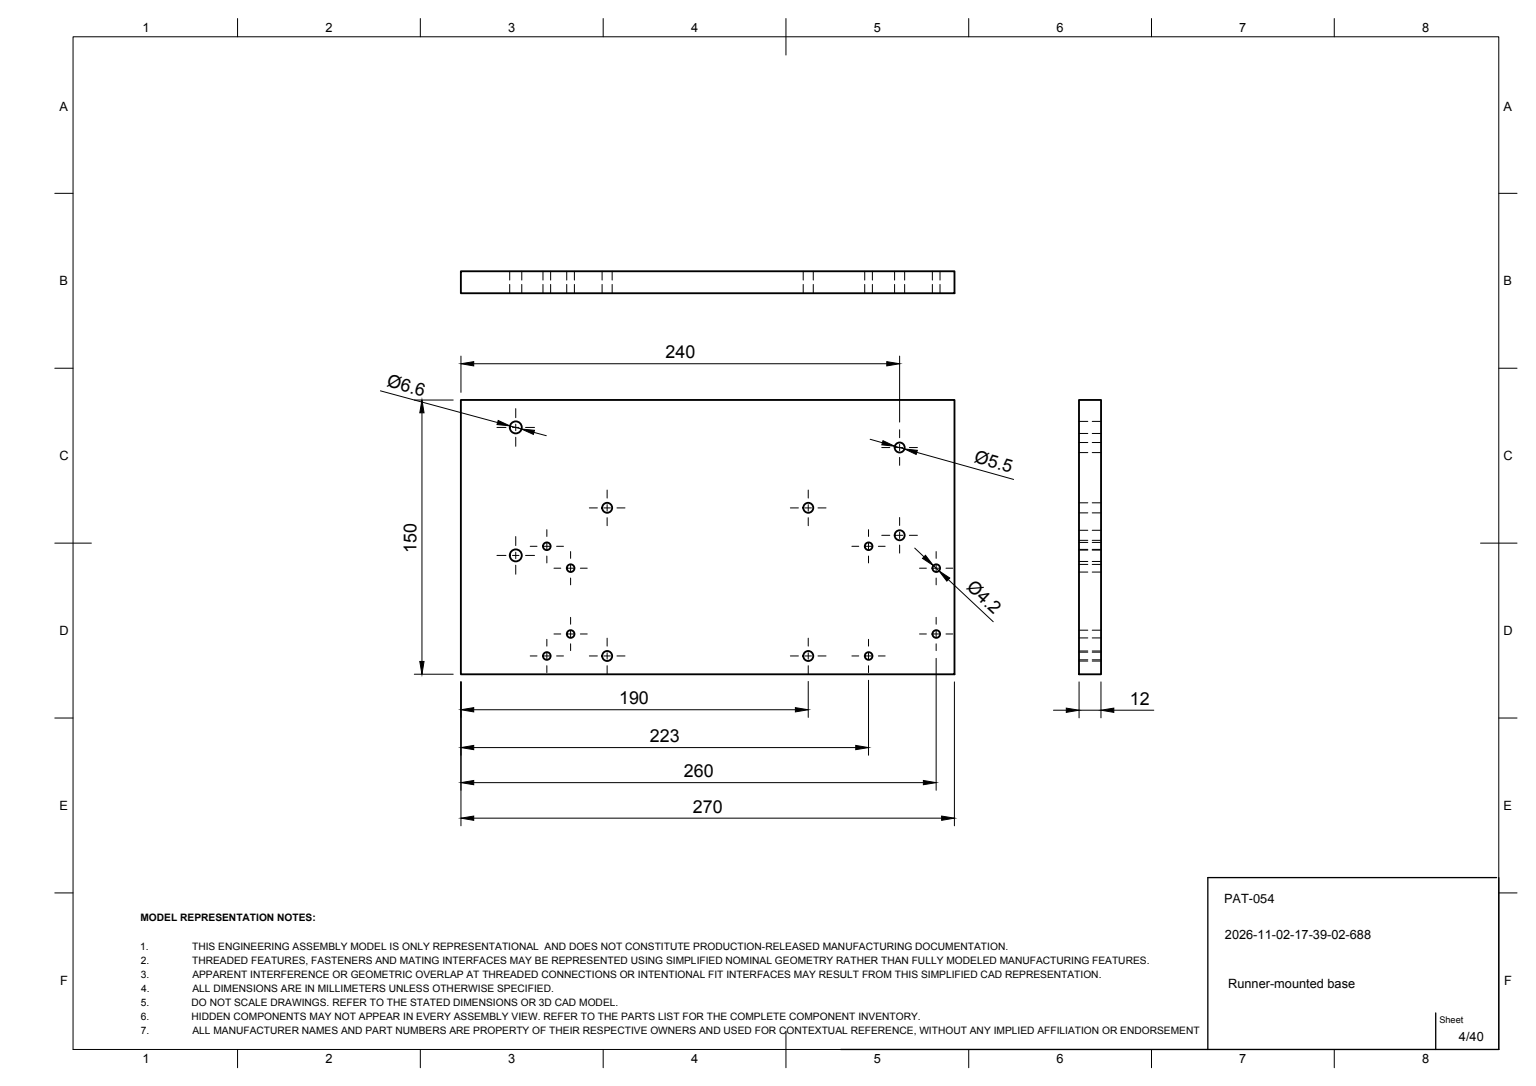
ISO-10303-21;
HEADER;
/* Generated by software containing ST-Developer
 * from STEP Tools, Inc. (www.steptools.com) 
 */

FILE_DESCRIPTION(
/* description */ ('PAT-054'),
/* implementation_level */ '2;1');

FILE_NAME(
/* name */ 'Runner-mounted base.step',
/* time_stamp */ '2026-10-29T16:38:13-07:00',
/* author */ (''),
/* organization */ (''),
/* preprocessor_version */ 'ST-DEVELOPER v20.2',
/* originating_system */ 'Autodesk Translation Framework v15.17.0.0',
/* authorisation */ '');

FILE_SCHEMA (('AUTOMOTIVE_DESIGN { 1 0 10303 214 3 1 1 }'));
ENDSEC;

DATA;
#10=MECHANICAL_DESIGN_GEOMETRIC_PRESENTATION_REPRESENTATION('',(#899),#33981);
#811=SHAPE_REPRESENTATION_RELATIONSHIP('SRR','None',#34184,#855);
#855=ADVANCED_BREP_SHAPE_REPRESENTATION('',(#958),#33932);
#899=STYLED_ITEM('',(#34496),#958);
#958=MANIFOLD_SOLID_BREP('Body1',#13010);
#1012=FACE_BOUND('',#2319,.T.);
#1013=FACE_BOUND('',#2320,.T.);
#1014=FACE_BOUND('',#2321,.T.);
#1015=FACE_BOUND('',#2322,.T.);
#1016=FACE_BOUND('',#2323,.T.);
#1017=FACE_BOUND('',#2324,.T.);
#1018=FACE_BOUND('',#2325,.T.);
#1019=FACE_BOUND('',#2326,.T.);
#1020=FACE_BOUND('',#2327,.T.);
#1021=FACE_BOUND('',#2328,.T.);
#1022=FACE_BOUND('',#2329,.T.);
#1023=FACE_BOUND('',#2330,.T.);
#1024=FACE_BOUND('',#2331,.T.);
#1025=FACE_BOUND('',#2332,.T.);
#1026=FACE_BOUND('',#2333,.T.);
#1027=FACE_BOUND('',#2334,.T.);
#1028=FACE_BOUND('',#2336,.T.);
#1029=FACE_BOUND('',#2337,.T.);
#1030=FACE_BOUND('',#2338,.T.);
#1031=FACE_BOUND('',#2339,.T.);
#1032=FACE_BOUND('',#2340,.T.);
#1033=FACE_BOUND('',#2341,.T.);
#1034=FACE_BOUND('',#2342,.T.);
#1035=FACE_BOUND('',#2343,.T.);
#1036=FACE_BOUND('',#2344,.T.);
#1037=FACE_BOUND('',#2345,.T.);
#1038=FACE_BOUND('',#2346,.T.);
#1039=FACE_BOUND('',#2347,.T.);
#1040=FACE_BOUND('',#2348,.T.);
#1041=FACE_BOUND('',#2349,.T.);
#1042=FACE_BOUND('',#2350,.T.);
#1043=FACE_BOUND('',#2351,.T.);
#1228=PLANE('',#13610);
#1229=PLANE('',#13611);
#1230=PLANE('',#13612);
#1231=PLANE('',#13613);
#1232=PLANE('',#13614);
#1233=PLANE('',#13615);
#1575=FACE_OUTER_BOUND('',#2298,.T.);
#1576=FACE_OUTER_BOUND('',#2299,.T.);
#1577=FACE_OUTER_BOUND('',#2300,.T.);
#1578=FACE_OUTER_BOUND('',#2301,.T.);
#1579=FACE_OUTER_BOUND('',#2302,.T.);
#1580=FACE_OUTER_BOUND('',#2303,.T.);
#1581=FACE_OUTER_BOUND('',#2304,.T.);
#1582=FACE_OUTER_BOUND('',#2305,.T.);
#1583=FACE_OUTER_BOUND('',#2306,.T.);
#1584=FACE_OUTER_BOUND('',#2307,.T.);
#1585=FACE_OUTER_BOUND('',#2308,.T.);
#1586=FACE_OUTER_BOUND('',#2309,.T.);
#1587=FACE_OUTER_BOUND('',#2310,.T.);
#1588=FACE_OUTER_BOUND('',#2311,.T.);
#1589=FACE_OUTER_BOUND('',#2312,.T.);
#1590=FACE_OUTER_BOUND('',#2313,.T.);
#1591=FACE_OUTER_BOUND('',#2314,.T.);
#1592=FACE_OUTER_BOUND('',#2315,.T.);
#1593=FACE_OUTER_BOUND('',#2316,.T.);
#1594=FACE_OUTER_BOUND('',#2317,.T.);
#1595=FACE_OUTER_BOUND('',#2318,.T.);
#1596=FACE_OUTER_BOUND('',#2335,.T.);
#2298=EDGE_LOOP('',(#8489,#8490,#8491,#8492));
#2299=EDGE_LOOP('',(#8493,#8494,#8495,#8496));
#2300=EDGE_LOOP('',(#8497,#8498,#8499,#8500));
#2301=EDGE_LOOP('',(#8501,#8502,#8503,#8504));
#2302=EDGE_LOOP('',(#8505,#8506,#8507,#8508));
#2303=EDGE_LOOP('',(#8509,#8510,#8511,#8512));
#2304=EDGE_LOOP('',(#8513,#8514,#8515,#8516));
#2305=EDGE_LOOP('',(#8517,#8518,#8519,#8520));
#2306=EDGE_LOOP('',(#8521,#8522,#8523,#8524));
#2307=EDGE_LOOP('',(#8525,#8526,#8527,#8528));
#2308=EDGE_LOOP('',(#8529,#8530,#8531,#8532));
#2309=EDGE_LOOP('',(#8533,#8534,#8535,#8536));
#2310=EDGE_LOOP('',(#8537,#8538,#8539,#8540));
#2311=EDGE_LOOP('',(#8541,#8542,#8543,#8544));
#2312=EDGE_LOOP('',(#8545,#8546,#8547,#8548));
#2313=EDGE_LOOP('',(#8549,#8550,#8551,#8552));
#2314=EDGE_LOOP('',(#8553,#8554,#8555,#8556));
#2315=EDGE_LOOP('',(#8557,#8558,#8559,#8560));
#2316=EDGE_LOOP('',(#8561,#8562,#8563,#8564));
#2317=EDGE_LOOP('',(#8565,#8566,#8567,#8568));
#2318=EDGE_LOOP('',(#8569,#8570,#8571,#8572));
#2319=EDGE_LOOP('',(#8573));
#2320=EDGE_LOOP('',(#8574));
#2321=EDGE_LOOP('',(#8575));
#2322=EDGE_LOOP('',(#8576));
#2323=EDGE_LOOP('',(#8577));
#2324=EDGE_LOOP('',(#8578));
#2325=EDGE_LOOP('',(#8579));
#2326=EDGE_LOOP('',(#8580));
#2327=EDGE_LOOP('',(#8581));
#2328=EDGE_LOOP('',(#8582));
#2329=EDGE_LOOP('',(#8583));
#2330=EDGE_LOOP('',(#8584));
#2331=EDGE_LOOP('',(#8585));
#2332=EDGE_LOOP('',(#8586));
#2333=EDGE_LOOP('',(#8587));
#2334=EDGE_LOOP('',(#8588));
#2335=EDGE_LOOP('',(#8589,#8590,#8591,#8592));
#2336=EDGE_LOOP('',(#8593));
#2337=EDGE_LOOP('',(#8594));
#2338=EDGE_LOOP('',(#8595));
#2339=EDGE_LOOP('',(#8596));
#2340=EDGE_LOOP('',(#8597));
#2341=EDGE_LOOP('',(#8598));
#2342=EDGE_LOOP('',(#8599));
#2343=EDGE_LOOP('',(#8600));
#2344=EDGE_LOOP('',(#8601));
#2345=EDGE_LOOP('',(#8602));
#2346=EDGE_LOOP('',(#8603));
#2347=EDGE_LOOP('',(#8604));
#2348=EDGE_LOOP('',(#8605));
#2349=EDGE_LOOP('',(#8606));
#2350=EDGE_LOOP('',(#8607));
#2351=EDGE_LOOP('',(#8608));
#3237=LINE('',#18493,#4171);
#3238=LINE('',#18499,#4172);
#3239=LINE('',#18505,#4173);
#3240=LINE('',#18511,#4174);
#3241=LINE('',#18517,#4175);
#3242=LINE('',#18523,#4176);
#3243=LINE('',#18529,#4177);
#3244=LINE('',#18535,#4178);
#3245=LINE('',#18541,#4179);
#3246=LINE('',#18547,#4180);
#3247=LINE('',#18553,#4181);
#3248=LINE('',#18559,#4182);
#3249=LINE('',#18565,#4183);
#3250=LINE('',#18571,#4184);
#3251=LINE('',#18577,#4185);
#3252=LINE('',#18583,#4186);
#3253=LINE('',#18588,#4187);
#3254=LINE('',#18590,#4188);
#3255=LINE('',#18592,#4189);
#3256=LINE('',#18593,#4190);
#3257=LINE('',#18596,#4191);
#3258=LINE('',#18598,#4192);
#3259=LINE('',#18599,#4193);
#3260=LINE('',#18602,#4194);
#3261=LINE('',#18604,#4195);
#3262=LINE('',#18605,#4196);
#3263=LINE('',#18607,#4197);
#3264=LINE('',#18608,#4198);
#4171=VECTOR('',#14900,0.274999999999999);
#4172=VECTOR('',#14907,0.275);
#4173=VECTOR('',#14914,0.275);
#4174=VECTOR('',#14921,0.274999999999999);
#4175=VECTOR('',#14928,0.210000000000001);
#4176=VECTOR('',#14935,0.210000000000001);
#4177=VECTOR('',#14942,0.21);
#4178=VECTOR('',#14949,0.21);
#4179=VECTOR('',#14956,0.329999999999998);
#4180=VECTOR('',#14963,0.329999999999998);
#4181=VECTOR('',#14970,0.275);
#4182=VECTOR('',#14977,0.275);
#4183=VECTOR('',#14984,0.210000000000001);
#4184=VECTOR('',#14991,0.21);
#4185=VECTOR('',#14998,0.21);
#4186=VECTOR('',#15005,0.210000000000001);
#4187=VECTOR('',#15010,1.);
#4188=VECTOR('',#15011,1.);
#4189=VECTOR('',#15012,1.);
#4190=VECTOR('',#15013,1.);
#4191=VECTOR('',#15016,1.);
#4192=VECTOR('',#15017,1.);
#4193=VECTOR('',#15018,1.);
#4194=VECTOR('',#15021,1.);
#4195=VECTOR('',#15022,1.);
#4196=VECTOR('',#15023,1.);
#4197=VECTOR('',#15026,1.);
#4198=VECTOR('',#15027,1.);
#5105=CIRCLE('',#13563,0.274999999999999);
#5106=CIRCLE('',#13564,0.274999999999999);
#5107=CIRCLE('',#13566,0.275);
#5108=CIRCLE('',#13567,0.275);
#5109=CIRCLE('',#13569,0.275);
#5110=CIRCLE('',#13570,0.275);
#5111=CIRCLE('',#13572,0.274999999999999);
#5112=CIRCLE('',#13573,0.274999999999999);
#5113=CIRCLE('',#13575,0.210000000000001);
#5114=CIRCLE('',#13576,0.210000000000001);
#5115=CIRCLE('',#13578,0.210000000000001);
#5116=CIRCLE('',#13579,0.210000000000001);
#5117=CIRCLE('',#13581,0.21);
#5118=CIRCLE('',#13582,0.21);
#5119=CIRCLE('',#13584,0.21);
#5120=CIRCLE('',#13585,0.21);
#5121=CIRCLE('',#13587,0.329999999999998);
#5122=CIRCLE('',#13588,0.329999999999998);
#5123=CIRCLE('',#13590,0.329999999999998);
#5124=CIRCLE('',#13591,0.329999999999998);
#5125=CIRCLE('',#13593,0.275);
#5126=CIRCLE('',#13594,0.275);
#5127=CIRCLE('',#13596,0.275);
#5128=CIRCLE('',#13597,0.275);
#5129=CIRCLE('',#13599,0.210000000000001);
#5130=CIRCLE('',#13600,0.210000000000001);
#5131=CIRCLE('',#13602,0.21);
#5132=CIRCLE('',#13603,0.21);
#5133=CIRCLE('',#13605,0.21);
#5134=CIRCLE('',#13606,0.21);
#5135=CIRCLE('',#13608,0.210000000000001);
#5136=CIRCLE('',#13609,0.210000000000001);
#5570=VERTEX_POINT('',#18490);
#5571=VERTEX_POINT('',#18492);
#5572=VERTEX_POINT('',#18496);
#5573=VERTEX_POINT('',#18498);
#5574=VERTEX_POINT('',#18502);
#5575=VERTEX_POINT('',#18504);
#5576=VERTEX_POINT('',#18508);
#5577=VERTEX_POINT('',#18510);
#5578=VERTEX_POINT('',#18514);
#5579=VERTEX_POINT('',#18516);
#5580=VERTEX_POINT('',#18520);
#5581=VERTEX_POINT('',#18522);
#5582=VERTEX_POINT('',#18526);
#5583=VERTEX_POINT('',#18528);
#5584=VERTEX_POINT('',#18532);
#5585=VERTEX_POINT('',#18534);
#5586=VERTEX_POINT('',#18538);
#5587=VERTEX_POINT('',#18540);
#5588=VERTEX_POINT('',#18544);
#5589=VERTEX_POINT('',#18546);
#5590=VERTEX_POINT('',#18550);
#5591=VERTEX_POINT('',#18552);
#5592=VERTEX_POINT('',#18556);
#5593=VERTEX_POINT('',#18558);
#5594=VERTEX_POINT('',#18562);
#5595=VERTEX_POINT('',#18564);
#5596=VERTEX_POINT('',#18568);
#5597=VERTEX_POINT('',#18570);
#5598=VERTEX_POINT('',#18574);
#5599=VERTEX_POINT('',#18576);
#5600=VERTEX_POINT('',#18580);
#5601=VERTEX_POINT('',#18582);
#5602=VERTEX_POINT('',#18586);
#5603=VERTEX_POINT('',#18587);
#5604=VERTEX_POINT('',#18589);
#5605=VERTEX_POINT('',#18591);
#5606=VERTEX_POINT('',#18595);
#5607=VERTEX_POINT('',#18597);
#5608=VERTEX_POINT('',#18601);
#5609=VERTEX_POINT('',#18603);
#6744=EDGE_CURVE('',#5570,#5570,#5105,.T.);
#6745=EDGE_CURVE('',#5570,#5571,#3237,.T.);
#6746=EDGE_CURVE('',#5571,#5571,#5106,.T.);
#6747=EDGE_CURVE('',#5572,#5572,#5107,.T.);
#6748=EDGE_CURVE('',#5572,#5573,#3238,.T.);
#6749=EDGE_CURVE('',#5573,#5573,#5108,.T.);
#6750=EDGE_CURVE('',#5574,#5574,#5109,.T.);
#6751=EDGE_CURVE('',#5574,#5575,#3239,.T.);
#6752=EDGE_CURVE('',#5575,#5575,#5110,.T.);
#6753=EDGE_CURVE('',#5576,#5576,#5111,.T.);
#6754=EDGE_CURVE('',#5576,#5577,#3240,.T.);
#6755=EDGE_CURVE('',#5577,#5577,#5112,.T.);
#6756=EDGE_CURVE('',#5578,#5578,#5113,.T.);
#6757=EDGE_CURVE('',#5578,#5579,#3241,.T.);
#6758=EDGE_CURVE('',#5579,#5579,#5114,.T.);
#6759=EDGE_CURVE('',#5580,#5580,#5115,.T.);
#6760=EDGE_CURVE('',#5580,#5581,#3242,.T.);
#6761=EDGE_CURVE('',#5581,#5581,#5116,.T.);
#6762=EDGE_CURVE('',#5582,#5582,#5117,.T.);
#6763=EDGE_CURVE('',#5582,#5583,#3243,.T.);
#6764=EDGE_CURVE('',#5583,#5583,#5118,.T.);
#6765=EDGE_CURVE('',#5584,#5584,#5119,.T.);
#6766=EDGE_CURVE('',#5584,#5585,#3244,.T.);
#6767=EDGE_CURVE('',#5585,#5585,#5120,.T.);
#6768=EDGE_CURVE('',#5586,#5586,#5121,.T.);
#6769=EDGE_CURVE('',#5586,#5587,#3245,.T.);
#6770=EDGE_CURVE('',#5587,#5587,#5122,.T.);
#6771=EDGE_CURVE('',#5588,#5588,#5123,.T.);
#6772=EDGE_CURVE('',#5588,#5589,#3246,.T.);
#6773=EDGE_CURVE('',#5589,#5589,#5124,.T.);
#6774=EDGE_CURVE('',#5590,#5590,#5125,.T.);
#6775=EDGE_CURVE('',#5590,#5591,#3247,.T.);
#6776=EDGE_CURVE('',#5591,#5591,#5126,.T.);
#6777=EDGE_CURVE('',#5592,#5592,#5127,.T.);
#6778=EDGE_CURVE('',#5592,#5593,#3248,.T.);
#6779=EDGE_CURVE('',#5593,#5593,#5128,.T.);
#6780=EDGE_CURVE('',#5594,#5594,#5129,.T.);
#6781=EDGE_CURVE('',#5594,#5595,#3249,.T.);
#6782=EDGE_CURVE('',#5595,#5595,#5130,.T.);
#6783=EDGE_CURVE('',#5596,#5596,#5131,.T.);
#6784=EDGE_CURVE('',#5596,#5597,#3250,.T.);
#6785=EDGE_CURVE('',#5597,#5597,#5132,.T.);
#6786=EDGE_CURVE('',#5598,#5598,#5133,.T.);
#6787=EDGE_CURVE('',#5598,#5599,#3251,.T.);
#6788=EDGE_CURVE('',#5599,#5599,#5134,.T.);
#6789=EDGE_CURVE('',#5600,#5600,#5135,.T.);
#6790=EDGE_CURVE('',#5600,#5601,#3252,.T.);
#6791=EDGE_CURVE('',#5601,#5601,#5136,.T.);
#6792=EDGE_CURVE('',#5602,#5603,#3253,.T.);
#6793=EDGE_CURVE('',#5603,#5604,#3254,.T.);
#6794=EDGE_CURVE('',#5605,#5604,#3255,.T.);
#6795=EDGE_CURVE('',#5602,#5605,#3256,.T.);
#6796=EDGE_CURVE('',#5606,#5602,#3257,.T.);
#6797=EDGE_CURVE('',#5607,#5605,#3258,.T.);
#6798=EDGE_CURVE('',#5606,#5607,#3259,.T.);
#6799=EDGE_CURVE('',#5608,#5606,#3260,.T.);
#6800=EDGE_CURVE('',#5609,#5607,#3261,.T.);
#6801=EDGE_CURVE('',#5608,#5609,#3262,.T.);
#6802=EDGE_CURVE('',#5603,#5608,#3263,.T.);
#6803=EDGE_CURVE('',#5604,#5609,#3264,.T.);
#8489=ORIENTED_EDGE('',*,*,#6744,.F.);
#8490=ORIENTED_EDGE('',*,*,#6745,.T.);
#8491=ORIENTED_EDGE('',*,*,#6746,.F.);
#8492=ORIENTED_EDGE('',*,*,#6745,.F.);
#8493=ORIENTED_EDGE('',*,*,#6747,.F.);
#8494=ORIENTED_EDGE('',*,*,#6748,.T.);
#8495=ORIENTED_EDGE('',*,*,#6749,.F.);
#8496=ORIENTED_EDGE('',*,*,#6748,.F.);
#8497=ORIENTED_EDGE('',*,*,#6750,.F.);
#8498=ORIENTED_EDGE('',*,*,#6751,.T.);
#8499=ORIENTED_EDGE('',*,*,#6752,.F.);
#8500=ORIENTED_EDGE('',*,*,#6751,.F.);
#8501=ORIENTED_EDGE('',*,*,#6753,.F.);
#8502=ORIENTED_EDGE('',*,*,#6754,.T.);
#8503=ORIENTED_EDGE('',*,*,#6755,.F.);
#8504=ORIENTED_EDGE('',*,*,#6754,.F.);
#8505=ORIENTED_EDGE('',*,*,#6756,.F.);
#8506=ORIENTED_EDGE('',*,*,#6757,.T.);
#8507=ORIENTED_EDGE('',*,*,#6758,.F.);
#8508=ORIENTED_EDGE('',*,*,#6757,.F.);
#8509=ORIENTED_EDGE('',*,*,#6759,.F.);
#8510=ORIENTED_EDGE('',*,*,#6760,.T.);
#8511=ORIENTED_EDGE('',*,*,#6761,.F.);
#8512=ORIENTED_EDGE('',*,*,#6760,.F.);
#8513=ORIENTED_EDGE('',*,*,#6762,.F.);
#8514=ORIENTED_EDGE('',*,*,#6763,.T.);
#8515=ORIENTED_EDGE('',*,*,#6764,.F.);
#8516=ORIENTED_EDGE('',*,*,#6763,.F.);
#8517=ORIENTED_EDGE('',*,*,#6765,.F.);
#8518=ORIENTED_EDGE('',*,*,#6766,.T.);
#8519=ORIENTED_EDGE('',*,*,#6767,.F.);
#8520=ORIENTED_EDGE('',*,*,#6766,.F.);
#8521=ORIENTED_EDGE('',*,*,#6768,.F.);
#8522=ORIENTED_EDGE('',*,*,#6769,.T.);
#8523=ORIENTED_EDGE('',*,*,#6770,.F.);
#8524=ORIENTED_EDGE('',*,*,#6769,.F.);
#8525=ORIENTED_EDGE('',*,*,#6771,.F.);
#8526=ORIENTED_EDGE('',*,*,#6772,.T.);
#8527=ORIENTED_EDGE('',*,*,#6773,.F.);
#8528=ORIENTED_EDGE('',*,*,#6772,.F.);
#8529=ORIENTED_EDGE('',*,*,#6774,.F.);
#8530=ORIENTED_EDGE('',*,*,#6775,.T.);
#8531=ORIENTED_EDGE('',*,*,#6776,.F.);
#8532=ORIENTED_EDGE('',*,*,#6775,.F.);
#8533=ORIENTED_EDGE('',*,*,#6777,.F.);
#8534=ORIENTED_EDGE('',*,*,#6778,.T.);
#8535=ORIENTED_EDGE('',*,*,#6779,.F.);
#8536=ORIENTED_EDGE('',*,*,#6778,.F.);
#8537=ORIENTED_EDGE('',*,*,#6780,.F.);
#8538=ORIENTED_EDGE('',*,*,#6781,.T.);
#8539=ORIENTED_EDGE('',*,*,#6782,.F.);
#8540=ORIENTED_EDGE('',*,*,#6781,.F.);
#8541=ORIENTED_EDGE('',*,*,#6783,.F.);
#8542=ORIENTED_EDGE('',*,*,#6784,.T.);
#8543=ORIENTED_EDGE('',*,*,#6785,.F.);
#8544=ORIENTED_EDGE('',*,*,#6784,.F.);
#8545=ORIENTED_EDGE('',*,*,#6786,.F.);
#8546=ORIENTED_EDGE('',*,*,#6787,.T.);
#8547=ORIENTED_EDGE('',*,*,#6788,.F.);
#8548=ORIENTED_EDGE('',*,*,#6787,.F.);
#8549=ORIENTED_EDGE('',*,*,#6789,.F.);
#8550=ORIENTED_EDGE('',*,*,#6790,.T.);
#8551=ORIENTED_EDGE('',*,*,#6791,.F.);
#8552=ORIENTED_EDGE('',*,*,#6790,.F.);
#8553=ORIENTED_EDGE('',*,*,#6792,.T.);
#8554=ORIENTED_EDGE('',*,*,#6793,.T.);
#8555=ORIENTED_EDGE('',*,*,#6794,.F.);
#8556=ORIENTED_EDGE('',*,*,#6795,.F.);
#8557=ORIENTED_EDGE('',*,*,#6796,.T.);
#8558=ORIENTED_EDGE('',*,*,#6795,.T.);
#8559=ORIENTED_EDGE('',*,*,#6797,.F.);
#8560=ORIENTED_EDGE('',*,*,#6798,.F.);
#8561=ORIENTED_EDGE('',*,*,#6799,.T.);
#8562=ORIENTED_EDGE('',*,*,#6798,.T.);
#8563=ORIENTED_EDGE('',*,*,#6800,.F.);
#8564=ORIENTED_EDGE('',*,*,#6801,.F.);
#8565=ORIENTED_EDGE('',*,*,#6802,.T.);
#8566=ORIENTED_EDGE('',*,*,#6801,.T.);
#8567=ORIENTED_EDGE('',*,*,#6803,.F.);
#8568=ORIENTED_EDGE('',*,*,#6793,.F.);
#8569=ORIENTED_EDGE('',*,*,#6803,.T.);
#8570=ORIENTED_EDGE('',*,*,#6800,.T.);
#8571=ORIENTED_EDGE('',*,*,#6797,.T.);
#8572=ORIENTED_EDGE('',*,*,#6794,.T.);
#8573=ORIENTED_EDGE('',*,*,#6758,.T.);
#8574=ORIENTED_EDGE('',*,*,#6761,.T.);
#8575=ORIENTED_EDGE('',*,*,#6770,.T.);
#8576=ORIENTED_EDGE('',*,*,#6773,.T.);
#8577=ORIENTED_EDGE('',*,*,#6776,.T.);
#8578=ORIENTED_EDGE('',*,*,#6779,.T.);
#8579=ORIENTED_EDGE('',*,*,#6782,.T.);
#8580=ORIENTED_EDGE('',*,*,#6785,.T.);
#8581=ORIENTED_EDGE('',*,*,#6788,.T.);
#8582=ORIENTED_EDGE('',*,*,#6791,.T.);
#8583=ORIENTED_EDGE('',*,*,#6767,.T.);
#8584=ORIENTED_EDGE('',*,*,#6764,.T.);
#8585=ORIENTED_EDGE('',*,*,#6755,.T.);
#8586=ORIENTED_EDGE('',*,*,#6752,.T.);
#8587=ORIENTED_EDGE('',*,*,#6749,.T.);
#8588=ORIENTED_EDGE('',*,*,#6746,.T.);
#8589=ORIENTED_EDGE('',*,*,#6802,.F.);
#8590=ORIENTED_EDGE('',*,*,#6792,.F.);
#8591=ORIENTED_EDGE('',*,*,#6796,.F.);
#8592=ORIENTED_EDGE('',*,*,#6799,.F.);
#8593=ORIENTED_EDGE('',*,*,#6756,.T.);
#8594=ORIENTED_EDGE('',*,*,#6759,.T.);
#8595=ORIENTED_EDGE('',*,*,#6768,.T.);
#8596=ORIENTED_EDGE('',*,*,#6771,.T.);
#8597=ORIENTED_EDGE('',*,*,#6774,.T.);
#8598=ORIENTED_EDGE('',*,*,#6777,.T.);
#8599=ORIENTED_EDGE('',*,*,#6780,.T.);
#8600=ORIENTED_EDGE('',*,*,#6783,.T.);
#8601=ORIENTED_EDGE('',*,*,#6786,.T.);
#8602=ORIENTED_EDGE('',*,*,#6789,.T.);
#8603=ORIENTED_EDGE('',*,*,#6765,.T.);
#8604=ORIENTED_EDGE('',*,*,#6762,.T.);
#8605=ORIENTED_EDGE('',*,*,#6753,.T.);
#8606=ORIENTED_EDGE('',*,*,#6750,.T.);
#8607=ORIENTED_EDGE('',*,*,#6747,.T.);
#8608=ORIENTED_EDGE('',*,*,#6744,.T.);
#11979=CYLINDRICAL_SURFACE('',#13562,0.274999999999999);
#11980=CYLINDRICAL_SURFACE('',#13565,0.275);
#11981=CYLINDRICAL_SURFACE('',#13568,0.275);
#11982=CYLINDRICAL_SURFACE('',#13571,0.274999999999999);
#11983=CYLINDRICAL_SURFACE('',#13574,0.210000000000001);
#11984=CYLINDRICAL_SURFACE('',#13577,0.210000000000001);
#11985=CYLINDRICAL_SURFACE('',#13580,0.21);
#11986=CYLINDRICAL_SURFACE('',#13583,0.21);
#11987=CYLINDRICAL_SURFACE('',#13586,0.329999999999998);
#11988=CYLINDRICAL_SURFACE('',#13589,0.329999999999998);
#11989=CYLINDRICAL_SURFACE('',#13592,0.275);
#11990=CYLINDRICAL_SURFACE('',#13595,0.275);
#11991=CYLINDRICAL_SURFACE('',#13598,0.210000000000001);
#11992=CYLINDRICAL_SURFACE('',#13601,0.21);
#11993=CYLINDRICAL_SURFACE('',#13604,0.21);
#11994=CYLINDRICAL_SURFACE('',#13607,0.210000000000001);
#12287=ADVANCED_FACE('',(#1575),#11979,.F.);
#12288=ADVANCED_FACE('',(#1576),#11980,.F.);
#12289=ADVANCED_FACE('',(#1577),#11981,.F.);
#12290=ADVANCED_FACE('',(#1578),#11982,.F.);
#12291=ADVANCED_FACE('',(#1579),#11983,.F.);
#12292=ADVANCED_FACE('',(#1580),#11984,.F.);
#12293=ADVANCED_FACE('',(#1581),#11985,.F.);
#12294=ADVANCED_FACE('',(#1582),#11986,.F.);
#12295=ADVANCED_FACE('',(#1583),#11987,.F.);
#12296=ADVANCED_FACE('',(#1584),#11988,.F.);
#12297=ADVANCED_FACE('',(#1585),#11989,.F.);
#12298=ADVANCED_FACE('',(#1586),#11990,.F.);
#12299=ADVANCED_FACE('',(#1587),#11991,.F.);
#12300=ADVANCED_FACE('',(#1588),#11992,.F.);
#12301=ADVANCED_FACE('',(#1589),#11993,.F.);
#12302=ADVANCED_FACE('',(#1590),#11994,.F.);
#12303=ADVANCED_FACE('',(#1591),#1228,.T.);
#12304=ADVANCED_FACE('',(#1592),#1229,.T.);
#12305=ADVANCED_FACE('',(#1593),#1230,.T.);
#12306=ADVANCED_FACE('',(#1594),#1231,.T.);
#12307=ADVANCED_FACE('',(#1595,#1012,#1013,#1014,#1015,#1016,#1017,#1018,
#1019,#1020,#1021,#1022,#1023,#1024,#1025,#1026,#1027),#1232,.T.);
#12308=ADVANCED_FACE('',(#1596,#1028,#1029,#1030,#1031,#1032,#1033,#1034,
#1035,#1036,#1037,#1038,#1039,#1040,#1041,#1042,#1043),#1233,.F.);
#13010=CLOSED_SHELL('',(#12287,#12288,#12289,#12290,#12291,#12292,#12293,
#12294,#12295,#12296,#12297,#12298,#12299,#12300,#12301,#12302,#12303,#12304,
#12305,#12306,#12307,#12308));
#13561=AXIS2_PLACEMENT_3D('',#18488,#14894,#14895);
#13562=AXIS2_PLACEMENT_3D('',#18489,#14896,#14897);
#13563=AXIS2_PLACEMENT_3D('',#18491,#14898,#14899);
#13564=AXIS2_PLACEMENT_3D('',#18494,#14901,#14902);
#13565=AXIS2_PLACEMENT_3D('',#18495,#14903,#14904);
#13566=AXIS2_PLACEMENT_3D('',#18497,#14905,#14906);
#13567=AXIS2_PLACEMENT_3D('',#18500,#14908,#14909);
#13568=AXIS2_PLACEMENT_3D('',#18501,#14910,#14911);
#13569=AXIS2_PLACEMENT_3D('',#18503,#14912,#14913);
#13570=AXIS2_PLACEMENT_3D('',#18506,#14915,#14916);
#13571=AXIS2_PLACEMENT_3D('',#18507,#14917,#14918);
#13572=AXIS2_PLACEMENT_3D('',#18509,#14919,#14920);
#13573=AXIS2_PLACEMENT_3D('',#18512,#14922,#14923);
#13574=AXIS2_PLACEMENT_3D('',#18513,#14924,#14925);
#13575=AXIS2_PLACEMENT_3D('',#18515,#14926,#14927);
#13576=AXIS2_PLACEMENT_3D('',#18518,#14929,#14930);
#13577=AXIS2_PLACEMENT_3D('',#18519,#14931,#14932);
#13578=AXIS2_PLACEMENT_3D('',#18521,#14933,#14934);
#13579=AXIS2_PLACEMENT_3D('',#18524,#14936,#14937);
#13580=AXIS2_PLACEMENT_3D('',#18525,#14938,#14939);
#13581=AXIS2_PLACEMENT_3D('',#18527,#14940,#14941);
#13582=AXIS2_PLACEMENT_3D('',#18530,#14943,#14944);
#13583=AXIS2_PLACEMENT_3D('',#18531,#14945,#14946);
#13584=AXIS2_PLACEMENT_3D('',#18533,#14947,#14948);
#13585=AXIS2_PLACEMENT_3D('',#18536,#14950,#14951);
#13586=AXIS2_PLACEMENT_3D('',#18537,#14952,#14953);
#13587=AXIS2_PLACEMENT_3D('',#18539,#14954,#14955);
#13588=AXIS2_PLACEMENT_3D('',#18542,#14957,#14958);
#13589=AXIS2_PLACEMENT_3D('',#18543,#14959,#14960);
#13590=AXIS2_PLACEMENT_3D('',#18545,#14961,#14962);
#13591=AXIS2_PLACEMENT_3D('',#18548,#14964,#14965);
#13592=AXIS2_PLACEMENT_3D('',#18549,#14966,#14967);
#13593=AXIS2_PLACEMENT_3D('',#18551,#14968,#14969);
#13594=AXIS2_PLACEMENT_3D('',#18554,#14971,#14972);
#13595=AXIS2_PLACEMENT_3D('',#18555,#14973,#14974);
#13596=AXIS2_PLACEMENT_3D('',#18557,#14975,#14976);
#13597=AXIS2_PLACEMENT_3D('',#18560,#14978,#14979);
#13598=AXIS2_PLACEMENT_3D('',#18561,#14980,#14981);
#13599=AXIS2_PLACEMENT_3D('',#18563,#14982,#14983);
#13600=AXIS2_PLACEMENT_3D('',#18566,#14985,#14986);
#13601=AXIS2_PLACEMENT_3D('',#18567,#14987,#14988);
#13602=AXIS2_PLACEMENT_3D('',#18569,#14989,#14990);
#13603=AXIS2_PLACEMENT_3D('',#18572,#14992,#14993);
#13604=AXIS2_PLACEMENT_3D('',#18573,#14994,#14995);
#13605=AXIS2_PLACEMENT_3D('',#18575,#14996,#14997);
#13606=AXIS2_PLACEMENT_3D('',#18578,#14999,#15000);
#13607=AXIS2_PLACEMENT_3D('',#18579,#15001,#15002);
#13608=AXIS2_PLACEMENT_3D('',#18581,#15003,#15004);
#13609=AXIS2_PLACEMENT_3D('',#18584,#15006,#15007);
#13610=AXIS2_PLACEMENT_3D('',#18585,#15008,#15009);
#13611=AXIS2_PLACEMENT_3D('',#18594,#15014,#15015);
#13612=AXIS2_PLACEMENT_3D('',#18600,#15019,#15020);
#13613=AXIS2_PLACEMENT_3D('',#18606,#15024,#15025);
#13614=AXIS2_PLACEMENT_3D('',#18609,#15028,#15029);
#13615=AXIS2_PLACEMENT_3D('',#18610,#15030,#15031);
#14894=DIRECTION('axis',(0.,0.,1.));
#14895=DIRECTION('refdir',(1.,0.,0.));
#14896=DIRECTION('center_axis',(0.,0.,1.));
#14897=DIRECTION('ref_axis',(1.,0.,0.));
#14898=DIRECTION('center_axis',(0.,0.,1.));
#14899=DIRECTION('ref_axis',(1.,0.,0.));
#14900=DIRECTION('',(0.,0.,1.));
#14901=DIRECTION('center_axis',(0.,0.,-1.));
#14902=DIRECTION('ref_axis',(1.,0.,0.));
#14903=DIRECTION('center_axis',(0.,0.,1.));
#14904=DIRECTION('ref_axis',(1.,0.,0.));
#14905=DIRECTION('center_axis',(0.,0.,1.));
#14906=DIRECTION('ref_axis',(1.,0.,0.));
#14907=DIRECTION('',(0.,0.,1.));
#14908=DIRECTION('center_axis',(0.,0.,-1.));
#14909=DIRECTION('ref_axis',(1.,0.,0.));
#14910=DIRECTION('center_axis',(0.,0.,1.));
#14911=DIRECTION('ref_axis',(1.,0.,0.));
#14912=DIRECTION('center_axis',(0.,0.,1.));
#14913=DIRECTION('ref_axis',(1.,0.,0.));
#14914=DIRECTION('',(0.,0.,1.));
#14915=DIRECTION('center_axis',(0.,0.,-1.));
#14916=DIRECTION('ref_axis',(1.,0.,0.));
#14917=DIRECTION('center_axis',(0.,0.,1.));
#14918=DIRECTION('ref_axis',(1.,0.,0.));
#14919=DIRECTION('center_axis',(0.,0.,1.));
#14920=DIRECTION('ref_axis',(1.,0.,0.));
#14921=DIRECTION('',(0.,0.,1.));
#14922=DIRECTION('center_axis',(0.,0.,-1.));
#14923=DIRECTION('ref_axis',(1.,0.,0.));
#14924=DIRECTION('center_axis',(0.,0.,1.));
#14925=DIRECTION('ref_axis',(1.,0.,0.));
#14926=DIRECTION('center_axis',(0.,0.,1.));
#14927=DIRECTION('ref_axis',(1.,0.,0.));
#14928=DIRECTION('',(0.,0.,1.));
#14929=DIRECTION('center_axis',(0.,0.,-1.));
#14930=DIRECTION('ref_axis',(1.,0.,0.));
#14931=DIRECTION('center_axis',(0.,0.,1.));
#14932=DIRECTION('ref_axis',(1.,0.,0.));
#14933=DIRECTION('center_axis',(0.,0.,1.));
#14934=DIRECTION('ref_axis',(1.,0.,0.));
#14935=DIRECTION('',(0.,0.,1.));
#14936=DIRECTION('center_axis',(0.,0.,-1.));
#14937=DIRECTION('ref_axis',(1.,0.,0.));
#14938=DIRECTION('center_axis',(0.,0.,1.));
#14939=DIRECTION('ref_axis',(1.,0.,0.));
#14940=DIRECTION('center_axis',(0.,0.,1.));
#14941=DIRECTION('ref_axis',(1.,0.,0.));
#14942=DIRECTION('',(0.,0.,1.));
#14943=DIRECTION('center_axis',(0.,0.,-1.));
#14944=DIRECTION('ref_axis',(1.,0.,0.));
#14945=DIRECTION('center_axis',(0.,0.,1.));
#14946=DIRECTION('ref_axis',(1.,0.,0.));
#14947=DIRECTION('center_axis',(0.,0.,1.));
#14948=DIRECTION('ref_axis',(1.,0.,0.));
#14949=DIRECTION('',(0.,0.,1.));
#14950=DIRECTION('center_axis',(0.,0.,-1.));
#14951=DIRECTION('ref_axis',(1.,0.,0.));
#14952=DIRECTION('center_axis',(0.,0.,1.));
#14953=DIRECTION('ref_axis',(1.,0.,0.));
#14954=DIRECTION('center_axis',(0.,0.,1.));
#14955=DIRECTION('ref_axis',(1.,0.,0.));
#14956=DIRECTION('',(0.,0.,1.));
#14957=DIRECTION('center_axis',(0.,0.,-1.));
#14958=DIRECTION('ref_axis',(1.,0.,0.));
#14959=DIRECTION('center_axis',(0.,0.,1.));
#14960=DIRECTION('ref_axis',(1.,0.,0.));
#14961=DIRECTION('center_axis',(0.,0.,1.));
#14962=DIRECTION('ref_axis',(1.,0.,0.));
#14963=DIRECTION('',(0.,0.,1.));
#14964=DIRECTION('center_axis',(0.,0.,-1.));
#14965=DIRECTION('ref_axis',(1.,0.,0.));
#14966=DIRECTION('center_axis',(0.,0.,1.));
#14967=DIRECTION('ref_axis',(1.,0.,0.));
#14968=DIRECTION('center_axis',(0.,0.,1.));
#14969=DIRECTION('ref_axis',(1.,0.,0.));
#14970=DIRECTION('',(0.,0.,1.));
#14971=DIRECTION('center_axis',(0.,0.,-1.));
#14972=DIRECTION('ref_axis',(1.,0.,0.));
#14973=DIRECTION('center_axis',(0.,0.,1.));
#14974=DIRECTION('ref_axis',(1.,0.,0.));
#14975=DIRECTION('center_axis',(0.,0.,1.));
#14976=DIRECTION('ref_axis',(1.,0.,0.));
#14977=DIRECTION('',(0.,0.,1.));
#14978=DIRECTION('center_axis',(0.,0.,-1.));
#14979=DIRECTION('ref_axis',(1.,0.,0.));
#14980=DIRECTION('center_axis',(0.,0.,1.));
#14981=DIRECTION('ref_axis',(1.,0.,0.));
#14982=DIRECTION('center_axis',(0.,0.,1.));
#14983=DIRECTION('ref_axis',(1.,0.,0.));
#14984=DIRECTION('',(0.,0.,1.));
#14985=DIRECTION('center_axis',(0.,0.,-1.));
#14986=DIRECTION('ref_axis',(1.,0.,0.));
#14987=DIRECTION('center_axis',(0.,0.,1.));
#14988=DIRECTION('ref_axis',(1.,0.,0.));
#14989=DIRECTION('center_axis',(0.,0.,1.));
#14990=DIRECTION('ref_axis',(1.,0.,0.));
#14991=DIRECTION('',(0.,0.,1.));
#14992=DIRECTION('center_axis',(0.,0.,-1.));
#14993=DIRECTION('ref_axis',(1.,0.,0.));
#14994=DIRECTION('center_axis',(0.,0.,1.));
#14995=DIRECTION('ref_axis',(1.,0.,0.));
#14996=DIRECTION('center_axis',(0.,0.,1.));
#14997=DIRECTION('ref_axis',(1.,0.,0.));
#14998=DIRECTION('',(0.,0.,1.));
#14999=DIRECTION('center_axis',(0.,0.,-1.));
#15000=DIRECTION('ref_axis',(1.,0.,0.));
#15001=DIRECTION('center_axis',(0.,0.,1.));
#15002=DIRECTION('ref_axis',(1.,0.,0.));
#15003=DIRECTION('center_axis',(0.,0.,1.));
#15004=DIRECTION('ref_axis',(1.,0.,0.));
#15005=DIRECTION('',(0.,0.,1.));
#15006=DIRECTION('center_axis',(0.,0.,-1.));
#15007=DIRECTION('ref_axis',(1.,0.,0.));
#15008=DIRECTION('center_axis',(0.,1.,0.));
#15009=DIRECTION('ref_axis',(-1.,0.,0.));
#15010=DIRECTION('',(-1.,0.,0.));
#15011=DIRECTION('',(0.,0.,1.));
#15012=DIRECTION('',(-1.,0.,0.));
#15013=DIRECTION('',(0.,0.,1.));
#15014=DIRECTION('center_axis',(1.,0.,0.));
#15015=DIRECTION('ref_axis',(0.,1.,0.));
#15016=DIRECTION('',(0.,1.,0.));
#15017=DIRECTION('',(0.,1.,0.));
#15018=DIRECTION('',(0.,0.,1.));
#15019=DIRECTION('center_axis',(0.,-1.,0.));
#15020=DIRECTION('ref_axis',(1.,0.,0.));
#15021=DIRECTION('',(1.,0.,0.));
#15022=DIRECTION('',(1.,0.,0.));
#15023=DIRECTION('',(0.,0.,1.));
#15024=DIRECTION('center_axis',(-1.,0.,0.));
#15025=DIRECTION('ref_axis',(0.,-1.,0.));
#15026=DIRECTION('',(0.,-1.,0.));
#15027=DIRECTION('',(0.,-1.,0.));
#15028=DIRECTION('center_axis',(0.,0.,1.));
#15029=DIRECTION('ref_axis',(1.,0.,0.));
#15030=DIRECTION('center_axis',(0.,0.,1.));
#15031=DIRECTION('ref_axis',(1.,0.,0.));
#18488=CARTESIAN_POINT('',(0.,0.,0.));
#18489=CARTESIAN_POINT('Origin',(19.,-9.,-0.1));
#18490=CARTESIAN_POINT('',(18.725,-9.,0.));
#18491=CARTESIAN_POINT('Origin',(19.,-9.,0.));
#18492=CARTESIAN_POINT('',(18.725,-9.,1.2));
#18493=CARTESIAN_POINT('',(18.725,-9.,-0.1));
#18494=CARTESIAN_POINT('Origin',(19.,-9.,1.2));
#18495=CARTESIAN_POINT('Origin',(8.,-0.9,-0.1));
#18496=CARTESIAN_POINT('',(7.725,-0.9,0.));
#18497=CARTESIAN_POINT('Origin',(8.,-0.9,0.));
#18498=CARTESIAN_POINT('',(7.725,-0.9,1.2));
#18499=CARTESIAN_POINT('',(7.725,-0.9,-0.1));
#18500=CARTESIAN_POINT('Origin',(8.,-0.9,1.2));
#18501=CARTESIAN_POINT('Origin',(8.,-9.,-0.1));
#18502=CARTESIAN_POINT('',(7.725,-9.,0.));
#18503=CARTESIAN_POINT('Origin',(8.,-9.,0.));
#18504=CARTESIAN_POINT('',(7.725,-9.,1.2));
#18505=CARTESIAN_POINT('',(7.725,-9.,-0.1));
#18506=CARTESIAN_POINT('Origin',(8.,-9.,1.2));
#18507=CARTESIAN_POINT('Origin',(19.,-0.9,-0.1));
#18508=CARTESIAN_POINT('',(18.725,-0.9,0.));
#18509=CARTESIAN_POINT('Origin',(19.,-0.9,0.));
#18510=CARTESIAN_POINT('',(18.725,-0.9,1.2));
#18511=CARTESIAN_POINT('',(18.725,-0.9,-0.1));
#18512=CARTESIAN_POINT('Origin',(19.,-0.9,1.2));
#18513=CARTESIAN_POINT('Origin',(22.3,-9.,-0.1));
#18514=CARTESIAN_POINT('',(22.09,-9.,0.));
#18515=CARTESIAN_POINT('Origin',(22.3,-9.,0.));
#18516=CARTESIAN_POINT('',(22.09,-9.,1.2));
#18517=CARTESIAN_POINT('',(22.09,-9.,-0.1));
#18518=CARTESIAN_POINT('Origin',(22.3,-9.,1.2));
#18519=CARTESIAN_POINT('Origin',(22.3,-3.,-0.1));
#18520=CARTESIAN_POINT('',(22.09,-3.,0.));
#18521=CARTESIAN_POINT('Origin',(22.3,-3.,0.));
#18522=CARTESIAN_POINT('',(22.09,-3.,1.2));
#18523=CARTESIAN_POINT('',(22.09,-3.,-0.1));
#18524=CARTESIAN_POINT('Origin',(22.3,-3.,1.2));
#18525=CARTESIAN_POINT('Origin',(4.7,-9.,-0.1));
#18526=CARTESIAN_POINT('',(4.49,-9.,0.));
#18527=CARTESIAN_POINT('Origin',(4.7,-9.,0.));
#18528=CARTESIAN_POINT('',(4.49,-9.,1.2));
#18529=CARTESIAN_POINT('',(4.49,-9.,-0.1));
#18530=CARTESIAN_POINT('Origin',(4.7,-9.,1.2));
#18531=CARTESIAN_POINT('Origin',(4.7,-3.,-0.1));
#18532=CARTESIAN_POINT('',(4.49,-3.,0.));
#18533=CARTESIAN_POINT('Origin',(4.7,-3.,0.));
#18534=CARTESIAN_POINT('',(4.49,-3.,1.2));
#18535=CARTESIAN_POINT('',(4.49,-3.,-0.1));
#18536=CARTESIAN_POINT('Origin',(4.7,-3.,1.2));
#18537=CARTESIAN_POINT('Origin',(24.,-3.5,-0.1));
#18538=CARTESIAN_POINT('',(23.67,-3.5,0.));
#18539=CARTESIAN_POINT('Origin',(24.,-3.5,0.));
#18540=CARTESIAN_POINT('',(23.67,-3.5,1.2));
#18541=CARTESIAN_POINT('',(23.67,-3.5,-0.1));
#18542=CARTESIAN_POINT('Origin',(24.,-3.5,1.2));
#18543=CARTESIAN_POINT('Origin',(24.,3.5,-0.1));
#18544=CARTESIAN_POINT('',(23.67,3.5,0.));
#18545=CARTESIAN_POINT('Origin',(24.,3.5,0.));
#18546=CARTESIAN_POINT('',(23.67,3.5,1.2));
#18547=CARTESIAN_POINT('',(23.67,3.5,-0.1));
#18548=CARTESIAN_POINT('Origin',(24.,3.5,1.2));
#18549=CARTESIAN_POINT('Origin',(3.,-2.4,-0.1));
#18550=CARTESIAN_POINT('',(2.725,-2.4,0.));
#18551=CARTESIAN_POINT('Origin',(3.,-2.4,0.));
#18552=CARTESIAN_POINT('',(2.725,-2.4,1.2));
#18553=CARTESIAN_POINT('',(2.725,-2.4,-0.1));
#18554=CARTESIAN_POINT('Origin',(3.,-2.4,1.2));
#18555=CARTESIAN_POINT('Origin',(3.,2.4,-0.1));
#18556=CARTESIAN_POINT('',(2.725,2.4,0.));
#18557=CARTESIAN_POINT('Origin',(3.,2.4,0.));
#18558=CARTESIAN_POINT('',(2.725,2.4,1.2));
#18559=CARTESIAN_POINT('',(2.725,2.4,-0.1));
#18560=CARTESIAN_POINT('Origin',(3.,2.4,1.2));
#18561=CARTESIAN_POINT('Origin',(21.,-7.8,-0.1));
#18562=CARTESIAN_POINT('',(20.79,-7.8,0.));
#18563=CARTESIAN_POINT('Origin',(21.,-7.8,0.));
#18564=CARTESIAN_POINT('',(20.79,-7.8,1.2));
#18565=CARTESIAN_POINT('',(20.79,-7.8,-0.1));
#18566=CARTESIAN_POINT('Origin',(21.,-7.8,1.2));
#18567=CARTESIAN_POINT('Origin',(1.,-4.2,-0.1));
#18568=CARTESIAN_POINT('',(0.79,-4.2,0.));
#18569=CARTESIAN_POINT('Origin',(1.,-4.2,0.));
#18570=CARTESIAN_POINT('',(0.79,-4.2,1.2));
#18571=CARTESIAN_POINT('',(0.79,-4.2,-0.1));
#18572=CARTESIAN_POINT('Origin',(1.,-4.2,1.2));
#18573=CARTESIAN_POINT('Origin',(1.,-7.8,-0.1));
#18574=CARTESIAN_POINT('',(0.79,-7.8,0.));
#18575=CARTESIAN_POINT('Origin',(1.,-7.8,0.));
#18576=CARTESIAN_POINT('',(0.79,-7.8,1.2));
#18577=CARTESIAN_POINT('',(0.79,-7.8,-0.1));
#18578=CARTESIAN_POINT('Origin',(1.,-7.8,1.2));
#18579=CARTESIAN_POINT('Origin',(21.,-4.2,-0.1));
#18580=CARTESIAN_POINT('',(20.79,-4.2,0.));
#18581=CARTESIAN_POINT('Origin',(21.,-4.2,0.));
#18582=CARTESIAN_POINT('',(20.79,-4.2,1.2));
#18583=CARTESIAN_POINT('',(20.79,-4.2,-0.1));
#18584=CARTESIAN_POINT('Origin',(21.,-4.2,1.2));
#18585=CARTESIAN_POINT('Origin',(27.,5.,0.));
#18586=CARTESIAN_POINT('',(27.,5.,0.));
#18587=CARTESIAN_POINT('',(0.,5.,0.));
#18588=CARTESIAN_POINT('',(27.,5.,0.));
#18589=CARTESIAN_POINT('',(0.,5.,1.2));
#18590=CARTESIAN_POINT('',(0.,5.,0.));
#18591=CARTESIAN_POINT('',(27.,5.,1.2));
#18592=CARTESIAN_POINT('',(27.,5.,1.2));
#18593=CARTESIAN_POINT('',(27.,5.,0.));
#18594=CARTESIAN_POINT('Origin',(27.,-10.,0.));
#18595=CARTESIAN_POINT('',(27.,-10.,0.));
#18596=CARTESIAN_POINT('',(27.,-10.,0.));
#18597=CARTESIAN_POINT('',(27.,-10.,1.2));
#18598=CARTESIAN_POINT('',(27.,-10.,1.2));
#18599=CARTESIAN_POINT('',(27.,-10.,0.));
#18600=CARTESIAN_POINT('Origin',(0.,-10.,0.));
#18601=CARTESIAN_POINT('',(0.,-10.,0.));
#18602=CARTESIAN_POINT('',(0.,-10.,0.));
#18603=CARTESIAN_POINT('',(0.,-10.,1.2));
#18604=CARTESIAN_POINT('',(0.,-10.,1.2));
#18605=CARTESIAN_POINT('',(0.,-10.,0.));
#18606=CARTESIAN_POINT('Origin',(0.,5.,0.));
#18607=CARTESIAN_POINT('',(0.,5.,0.));
#18608=CARTESIAN_POINT('',(0.,5.,1.2));
#18609=CARTESIAN_POINT('Origin',(13.5,-2.5,1.2));
#18610=CARTESIAN_POINT('Origin',(13.5,-2.5,0.));
#33880=UNCERTAINTY_MEASURE_WITH_UNIT(LENGTH_MEASURE(0.001),#33982,
'DISTANCE_ACCURACY_VALUE',
'Maximum model space distance between geometric entities at asserted c
onnectivities');
#33929=UNCERTAINTY_MEASURE_WITH_UNIT(LENGTH_MEASURE(0.001),#33982,
'DISTANCE_ACCURACY_VALUE',
'Maximum model space distance between geometric entities at asserted c
onnectivities');
#33932=(
GEOMETRIC_REPRESENTATION_CONTEXT(3)
GLOBAL_UNCERTAINTY_ASSIGNED_CONTEXT((#33880))
GLOBAL_UNIT_ASSIGNED_CONTEXT((#33982,#33984,#33985))
REPRESENTATION_CONTEXT('','3D')
);
#33981=(
GEOMETRIC_REPRESENTATION_CONTEXT(3)
GLOBAL_UNCERTAINTY_ASSIGNED_CONTEXT((#33929))
GLOBAL_UNIT_ASSIGNED_CONTEXT((#33982,#33984,#33985))
REPRESENTATION_CONTEXT('','3D')
);
#33982=(
LENGTH_UNIT()
NAMED_UNIT(*)
SI_UNIT(.CENTI.,.METRE.)
);
#33984=(
NAMED_UNIT(*)
PLANE_ANGLE_UNIT()
SI_UNIT($,.RADIAN.)
);
#33985=(
NAMED_UNIT(*)
SI_UNIT($,.STERADIAN.)
SOLID_ANGLE_UNIT()
);
#33988=SHAPE_DEFINITION_REPRESENTATION(#34039,#34184);
#34039=PRODUCT_DEFINITION_SHAPE('',$,#34236);
#34184=SHAPE_REPRESENTATION('',(#13561),#33932);
#34233=PRODUCT_DEFINITION_CONTEXT('part definition',#34388,'design');
#34236=PRODUCT_DEFINITION('Runner-mounted base','Runner-mounted base',#34287,
#34233);
#34287=PRODUCT_DEFINITION_FORMATION('',$,#34392);
#34388=APPLICATION_CONTEXT(
'Core Data for Automotive Mechanical Design Process');
#34389=PRODUCT_CONTEXT('part definition',#34388,'mechanical');
#34392=PRODUCT('Runner-mounted base','Runner-mounted base',
'Runner-mounted base',(#34389));
#34490=COLOUR_RGB('Dark Blue',0.08,0.2,0.34);
#34491=FILL_AREA_STYLE_COLOUR('',#34490);
#34492=FILL_AREA_STYLE('',(#34491));
#34493=SURFACE_STYLE_FILL_AREA(#34492);
#34494=SURFACE_SIDE_STYLE('',(#34493));
#34495=SURFACE_STYLE_USAGE(.BOTH.,#34494);
#34496=PRESENTATION_STYLE_ASSIGNMENT((#34495));
ENDSEC;
END-ISO-10303-21;
